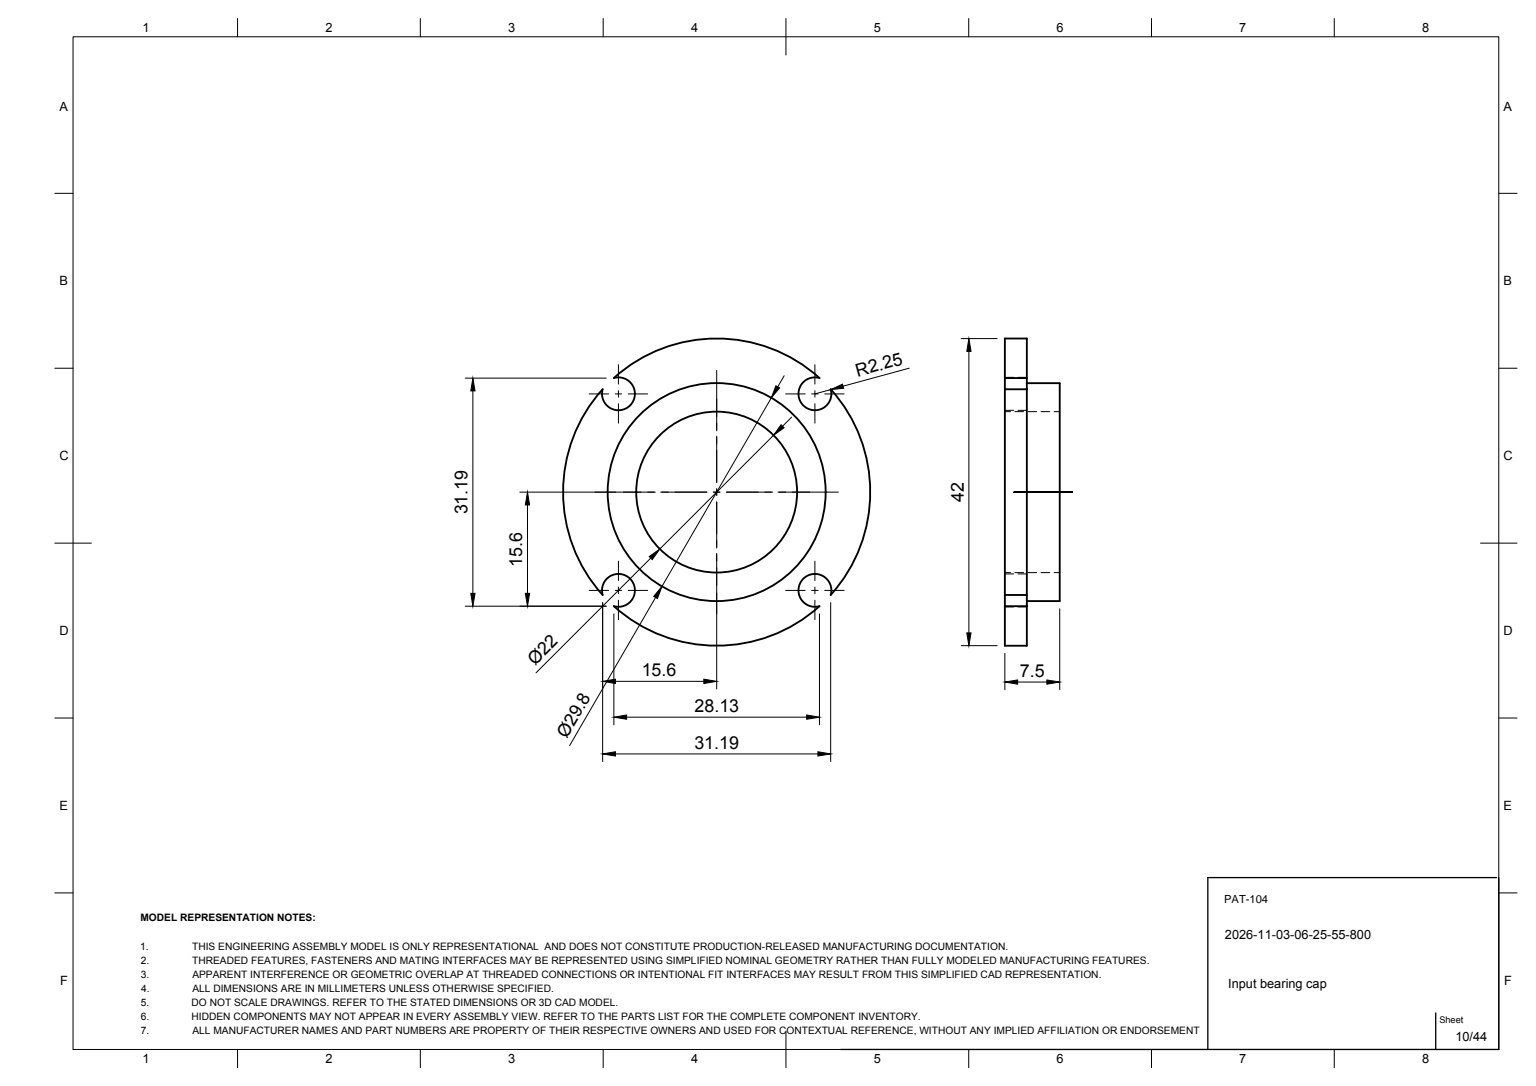
ISO-10303-21;
HEADER;
/* Generated by software containing ST-Developer
 * from STEP Tools, Inc. (www.steptools.com) 
 */

FILE_DESCRIPTION(
/* description */ ('Timing belt drive module 2 mm Pitch Timing 20T-40T'),

/* implementation_level */ '2;1');

FILE_NAME(
/* name */ 'Input bearing cap.step',
/* time_stamp */ '2026-10-28T03:25:12-07:00',
/* author */ (''),
/* organization */ (''),
/* preprocessor_version */ 'ST-DEVELOPER v20.2',
/* originating_system */ 'Autodesk Translation Framework v15.17.0.0',
/* authorisation */ '');

FILE_SCHEMA (('AUTOMOTIVE_DESIGN { 1 0 10303 214 3 1 1 }'));
ENDSEC;

DATA;
#10=MECHANICAL_DESIGN_GEOMETRIC_PRESENTATION_REPRESENTATION('',(#529),#17830);
#443=SHAPE_REPRESENTATION_RELATIONSHIP('SRR','None',#18013,#486);
#486=ADVANCED_BREP_SHAPE_REPRESENTATION('',(#587),#17788);
#529=STYLED_ITEM('',(#18317),#587);
#587=MANIFOLD_SOLID_BREP('Body1',#8986);
#667=FACE_BOUND('',#1583,.T.);
#668=FACE_BOUND('',#1590,.T.);
#669=FACE_BOUND('',#1593,.T.);
#815=PLANE('',#9651);
#816=PLANE('',#9668);
#817=PLANE('',#9671);
#1027=FACE_OUTER_BOUND('',#1578,.T.);
#1028=FACE_OUTER_BOUND('',#1579,.T.);
#1029=FACE_OUTER_BOUND('',#1580,.T.);
#1030=FACE_OUTER_BOUND('',#1581,.T.);
#1031=FACE_OUTER_BOUND('',#1582,.T.);
#1032=FACE_OUTER_BOUND('',#1584,.T.);
#1033=FACE_OUTER_BOUND('',#1585,.T.);
#1034=FACE_OUTER_BOUND('',#1586,.T.);
#1035=FACE_OUTER_BOUND('',#1587,.T.);
#1036=FACE_OUTER_BOUND('',#1588,.T.);
#1037=FACE_OUTER_BOUND('',#1589,.T.);
#1038=FACE_OUTER_BOUND('',#1591,.T.);
#1039=FACE_OUTER_BOUND('',#1592,.T.);
#1578=EDGE_LOOP('',(#6091,#6092,#6093,#6094));
#1579=EDGE_LOOP('',(#6095,#6096,#6097,#6098));
#1580=EDGE_LOOP('',(#6099,#6100,#6101,#6102));
#1581=EDGE_LOOP('',(#6103,#6104,#6105,#6106));
#1582=EDGE_LOOP('',(#6107,#6108,#6109,#6110,#6111,#6112,#6113,#6114));
#1583=EDGE_LOOP('',(#6115));
#1584=EDGE_LOOP('',(#6116,#6117,#6118,#6119));
#1585=EDGE_LOOP('',(#6120,#6121,#6122,#6123));
#1586=EDGE_LOOP('',(#6124,#6125,#6126,#6127));
#1587=EDGE_LOOP('',(#6128,#6129,#6130,#6131));
#1588=EDGE_LOOP('',(#6132,#6133,#6134,#6135));
#1589=EDGE_LOOP('',(#6136));
#1590=EDGE_LOOP('',(#6137));
#1591=EDGE_LOOP('',(#6138,#6139,#6140,#6141));
#1592=EDGE_LOOP('',(#6142,#6143,#6144,#6145,#6146,#6147,#6148,#6149));
#1593=EDGE_LOOP('',(#6150));
#2190=CIRCLE('',#9640,0.225);
#2191=CIRCLE('',#9641,0.225);
#2192=CIRCLE('',#9643,0.225);
#2193=CIRCLE('',#9644,0.225);
#2194=CIRCLE('',#9646,0.225);
#2195=CIRCLE('',#9647,0.225);
#2196=CIRCLE('',#9649,0.225);
#2197=CIRCLE('',#9650,0.225);
#2198=CIRCLE('',#9652,2.1);
#2199=CIRCLE('',#9653,2.1);
#2200=CIRCLE('',#9654,2.1);
#2201=CIRCLE('',#9655,2.1);
#2202=CIRCLE('',#9656,1.1);
#2203=CIRCLE('',#9658,2.1);
#2204=CIRCLE('',#9660,2.1);
#2205=CIRCLE('',#9662,2.1);
#2206=CIRCLE('',#9664,2.1);
#2207=CIRCLE('',#9666,1.49);
#2208=CIRCLE('',#9667,1.49);
#2209=CIRCLE('',#9669,1.1);
#2899=LINE('',#14214,#3377);
#2900=LINE('',#14218,#3378);
#2901=LINE('',#14223,#3379);
#2902=LINE('',#14227,#3380);
#2903=LINE('',#14232,#3381);
#2904=LINE('',#14236,#3382);
#2905=LINE('',#14241,#3383);
#2906=LINE('',#14245,#3384);
#2907=LINE('',#14266,#3385);
#2908=LINE('',#14272,#3386);
#3377=VECTOR('',#11166,1.);
#3378=VECTOR('',#11169,1.);
#3379=VECTOR('',#11174,1.);
#3380=VECTOR('',#11177,1.);
#3381=VECTOR('',#11182,1.);
#3382=VECTOR('',#11185,1.);
#3383=VECTOR('',#11190,1.);
#3384=VECTOR('',#11193,1.);
#3385=VECTOR('',#11228,1.49);
#3386=VECTOR('',#11237,1.1);
#3852=VERTEX_POINT('',#14212);
#3853=VERTEX_POINT('',#14213);
#3854=VERTEX_POINT('',#14215);
#3855=VERTEX_POINT('',#14217);
#3856=VERTEX_POINT('',#14221);
#3857=VERTEX_POINT('',#14222);
#3858=VERTEX_POINT('',#14224);
#3859=VERTEX_POINT('',#14226);
#3860=VERTEX_POINT('',#14230);
#3861=VERTEX_POINT('',#14231);
#3862=VERTEX_POINT('',#14233);
#3863=VERTEX_POINT('',#14235);
#3864=VERTEX_POINT('',#14239);
#3865=VERTEX_POINT('',#14240);
#3866=VERTEX_POINT('',#14242);
#3867=VERTEX_POINT('',#14244);
#3868=VERTEX_POINT('',#14252);
#3869=VERTEX_POINT('',#14263);
#3870=VERTEX_POINT('',#14265);
#3871=VERTEX_POINT('',#14269);
#4728=EDGE_CURVE('',#3852,#3853,#2899,.T.);
#4729=EDGE_CURVE('',#3854,#3852,#2190,.T.);
#4730=EDGE_CURVE('',#3855,#3854,#2900,.T.);
#4731=EDGE_CURVE('',#3853,#3855,#2191,.T.);
#4732=EDGE_CURVE('',#3856,#3857,#2901,.T.);
#4733=EDGE_CURVE('',#3858,#3856,#2192,.T.);
#4734=EDGE_CURVE('',#3859,#3858,#2902,.T.);
#4735=EDGE_CURVE('',#3857,#3859,#2193,.T.);
#4736=EDGE_CURVE('',#3860,#3861,#2903,.T.);
#4737=EDGE_CURVE('',#3862,#3860,#2194,.T.);
#4738=EDGE_CURVE('',#3863,#3862,#2904,.T.);
#4739=EDGE_CURVE('',#3861,#3863,#2195,.T.);
#4740=EDGE_CURVE('',#3864,#3865,#2905,.T.);
#4741=EDGE_CURVE('',#3866,#3864,#2196,.T.);
#4742=EDGE_CURVE('',#3867,#3866,#2906,.T.);
#4743=EDGE_CURVE('',#3865,#3867,#2197,.T.);
#4744=EDGE_CURVE('',#3866,#3852,#2198,.T.);
#4745=EDGE_CURVE('',#3862,#3864,#2199,.T.);
#4746=EDGE_CURVE('',#3858,#3860,#2200,.T.);
#4747=EDGE_CURVE('',#3854,#3856,#2201,.T.);
#4748=EDGE_CURVE('',#3868,#3868,#2202,.T.);
#4749=EDGE_CURVE('',#3863,#3865,#2203,.T.);
#4750=EDGE_CURVE('',#3859,#3861,#2204,.T.);
#4751=EDGE_CURVE('',#3867,#3853,#2205,.T.);
#4752=EDGE_CURVE('',#3855,#3857,#2206,.T.);
#4753=EDGE_CURVE('',#3869,#3869,#2207,.T.);
#4754=EDGE_CURVE('',#3869,#3870,#2907,.T.);
#4755=EDGE_CURVE('',#3870,#3870,#2208,.T.);
#4756=EDGE_CURVE('',#3871,#3871,#2209,.T.);
#4757=EDGE_CURVE('',#3871,#3868,#2908,.T.);
#6091=ORIENTED_EDGE('',*,*,#4728,.F.);
#6092=ORIENTED_EDGE('',*,*,#4729,.F.);
#6093=ORIENTED_EDGE('',*,*,#4730,.F.);
#6094=ORIENTED_EDGE('',*,*,#4731,.F.);
#6095=ORIENTED_EDGE('',*,*,#4732,.F.);
#6096=ORIENTED_EDGE('',*,*,#4733,.F.);
#6097=ORIENTED_EDGE('',*,*,#4734,.F.);
#6098=ORIENTED_EDGE('',*,*,#4735,.F.);
#6099=ORIENTED_EDGE('',*,*,#4736,.F.);
#6100=ORIENTED_EDGE('',*,*,#4737,.F.);
#6101=ORIENTED_EDGE('',*,*,#4738,.F.);
#6102=ORIENTED_EDGE('',*,*,#4739,.F.);
#6103=ORIENTED_EDGE('',*,*,#4740,.F.);
#6104=ORIENTED_EDGE('',*,*,#4741,.F.);
#6105=ORIENTED_EDGE('',*,*,#4742,.F.);
#6106=ORIENTED_EDGE('',*,*,#4743,.F.);
#6107=ORIENTED_EDGE('',*,*,#4729,.T.);
#6108=ORIENTED_EDGE('',*,*,#4744,.F.);
#6109=ORIENTED_EDGE('',*,*,#4741,.T.);
#6110=ORIENTED_EDGE('',*,*,#4745,.F.);
#6111=ORIENTED_EDGE('',*,*,#4737,.T.);
#6112=ORIENTED_EDGE('',*,*,#4746,.F.);
#6113=ORIENTED_EDGE('',*,*,#4733,.T.);
#6114=ORIENTED_EDGE('',*,*,#4747,.F.);
#6115=ORIENTED_EDGE('',*,*,#4748,.F.);
#6116=ORIENTED_EDGE('',*,*,#4738,.T.);
#6117=ORIENTED_EDGE('',*,*,#4745,.T.);
#6118=ORIENTED_EDGE('',*,*,#4740,.T.);
#6119=ORIENTED_EDGE('',*,*,#4749,.F.);
#6120=ORIENTED_EDGE('',*,*,#4734,.T.);
#6121=ORIENTED_EDGE('',*,*,#4746,.T.);
#6122=ORIENTED_EDGE('',*,*,#4736,.T.);
#6123=ORIENTED_EDGE('',*,*,#4750,.F.);
#6124=ORIENTED_EDGE('',*,*,#4728,.T.);
#6125=ORIENTED_EDGE('',*,*,#4751,.F.);
#6126=ORIENTED_EDGE('',*,*,#4742,.T.);
#6127=ORIENTED_EDGE('',*,*,#4744,.T.);
#6128=ORIENTED_EDGE('',*,*,#4730,.T.);
#6129=ORIENTED_EDGE('',*,*,#4747,.T.);
#6130=ORIENTED_EDGE('',*,*,#4732,.T.);
#6131=ORIENTED_EDGE('',*,*,#4752,.F.);
#6132=ORIENTED_EDGE('',*,*,#4753,.F.);
#6133=ORIENTED_EDGE('',*,*,#4754,.T.);
#6134=ORIENTED_EDGE('',*,*,#4755,.F.);
#6135=ORIENTED_EDGE('',*,*,#4754,.F.);
#6136=ORIENTED_EDGE('',*,*,#4753,.T.);
#6137=ORIENTED_EDGE('',*,*,#4756,.T.);
#6138=ORIENTED_EDGE('',*,*,#4756,.F.);
#6139=ORIENTED_EDGE('',*,*,#4757,.T.);
#6140=ORIENTED_EDGE('',*,*,#4748,.T.);
#6141=ORIENTED_EDGE('',*,*,#4757,.F.);
#6142=ORIENTED_EDGE('',*,*,#4731,.T.);
#6143=ORIENTED_EDGE('',*,*,#4752,.T.);
#6144=ORIENTED_EDGE('',*,*,#4735,.T.);
#6145=ORIENTED_EDGE('',*,*,#4750,.T.);
#6146=ORIENTED_EDGE('',*,*,#4739,.T.);
#6147=ORIENTED_EDGE('',*,*,#4749,.T.);
#6148=ORIENTED_EDGE('',*,*,#4743,.T.);
#6149=ORIENTED_EDGE('',*,*,#4751,.T.);
#6150=ORIENTED_EDGE('',*,*,#4755,.T.);
#8204=CYLINDRICAL_SURFACE('',#9639,0.225);
#8205=CYLINDRICAL_SURFACE('',#9642,0.225);
#8206=CYLINDRICAL_SURFACE('',#9645,0.225);
#8207=CYLINDRICAL_SURFACE('',#9648,0.225);
#8208=CYLINDRICAL_SURFACE('',#9657,2.1);
#8209=CYLINDRICAL_SURFACE('',#9659,2.1);
#8210=CYLINDRICAL_SURFACE('',#9661,2.1);
#8211=CYLINDRICAL_SURFACE('',#9663,2.1);
#8212=CYLINDRICAL_SURFACE('',#9665,1.49);
#8213=CYLINDRICAL_SURFACE('',#9670,1.1);
#8525=ADVANCED_FACE('',(#1027),#8204,.F.);
#8526=ADVANCED_FACE('',(#1028),#8205,.F.);
#8527=ADVANCED_FACE('',(#1029),#8206,.F.);
#8528=ADVANCED_FACE('',(#1030),#8207,.F.);
#8529=ADVANCED_FACE('',(#1031,#667),#815,.F.);
#8530=ADVANCED_FACE('',(#1032),#8208,.T.);
#8531=ADVANCED_FACE('',(#1033),#8209,.T.);
#8532=ADVANCED_FACE('',(#1034),#8210,.T.);
#8533=ADVANCED_FACE('',(#1035),#8211,.T.);
#8534=ADVANCED_FACE('',(#1036),#8212,.T.);
#8535=ADVANCED_FACE('',(#1037,#668),#816,.T.);
#8536=ADVANCED_FACE('',(#1038),#8213,.F.);
#8537=ADVANCED_FACE('',(#1039,#669),#817,.T.);
#8986=CLOSED_SHELL('',(#8525,#8526,#8527,#8528,#8529,#8530,#8531,#8532,
#8533,#8534,#8535,#8536,#8537));
#9638=AXIS2_PLACEMENT_3D('',#14210,#11162,#11163);
#9639=AXIS2_PLACEMENT_3D('',#14211,#11164,#11165);
#9640=AXIS2_PLACEMENT_3D('',#14216,#11167,#11168);
#9641=AXIS2_PLACEMENT_3D('',#14219,#11170,#11171);
#9642=AXIS2_PLACEMENT_3D('',#14220,#11172,#11173);
#9643=AXIS2_PLACEMENT_3D('',#14225,#11175,#11176);
#9644=AXIS2_PLACEMENT_3D('',#14228,#11178,#11179);
#9645=AXIS2_PLACEMENT_3D('',#14229,#11180,#11181);
#9646=AXIS2_PLACEMENT_3D('',#14234,#11183,#11184);
#9647=AXIS2_PLACEMENT_3D('',#14237,#11186,#11187);
#9648=AXIS2_PLACEMENT_3D('',#14238,#11188,#11189);
#9649=AXIS2_PLACEMENT_3D('',#14243,#11191,#11192);
#9650=AXIS2_PLACEMENT_3D('',#14246,#11194,#11195);
#9651=AXIS2_PLACEMENT_3D('',#14247,#11196,#11197);
#9652=AXIS2_PLACEMENT_3D('',#14248,#11198,#11199);
#9653=AXIS2_PLACEMENT_3D('',#14249,#11200,#11201);
#9654=AXIS2_PLACEMENT_3D('',#14250,#11202,#11203);
#9655=AXIS2_PLACEMENT_3D('',#14251,#11204,#11205);
#9656=AXIS2_PLACEMENT_3D('',#14253,#11206,#11207);
#9657=AXIS2_PLACEMENT_3D('',#14254,#11208,#11209);
#9658=AXIS2_PLACEMENT_3D('',#14255,#11210,#11211);
#9659=AXIS2_PLACEMENT_3D('',#14256,#11212,#11213);
#9660=AXIS2_PLACEMENT_3D('',#14257,#11214,#11215);
#9661=AXIS2_PLACEMENT_3D('',#14258,#11216,#11217);
#9662=AXIS2_PLACEMENT_3D('',#14259,#11218,#11219);
#9663=AXIS2_PLACEMENT_3D('',#14260,#11220,#11221);
#9664=AXIS2_PLACEMENT_3D('',#14261,#11222,#11223);
#9665=AXIS2_PLACEMENT_3D('',#14262,#11224,#11225);
#9666=AXIS2_PLACEMENT_3D('',#14264,#11226,#11227);
#9667=AXIS2_PLACEMENT_3D('',#14267,#11229,#11230);
#9668=AXIS2_PLACEMENT_3D('',#14268,#11231,#11232);
#9669=AXIS2_PLACEMENT_3D('',#14270,#11233,#11234);
#9670=AXIS2_PLACEMENT_3D('',#14271,#11235,#11236);
#9671=AXIS2_PLACEMENT_3D('',#14273,#11238,#11239);
#11162=DIRECTION('axis',(0.,0.,1.));
#11163=DIRECTION('refdir',(1.,0.,0.));
#11164=DIRECTION('center_axis',(0.,1.,0.));
#11165=DIRECTION('ref_axis',(0.707106781186546,0.,0.707106781186549));
#11166=DIRECTION('',(0.,1.,0.));
#11167=DIRECTION('center_axis',(0.,1.,0.));
#11168=DIRECTION('ref_axis',(1.,0.,0.));
#11169=DIRECTION('',(0.,-1.,0.));
#11170=DIRECTION('center_axis',(0.,-1.,0.));
#11171=DIRECTION('ref_axis',(1.,0.,0.));
#11172=DIRECTION('center_axis',(0.,1.,0.));
#11173=DIRECTION('ref_axis',(0.707106781186547,0.,-0.707106781186548));
#11174=DIRECTION('',(0.,1.,0.));
#11175=DIRECTION('center_axis',(0.,1.,0.));
#11176=DIRECTION('ref_axis',(1.,0.,0.));
#11177=DIRECTION('',(0.,-1.,0.));
#11178=DIRECTION('center_axis',(0.,-1.,0.));
#11179=DIRECTION('ref_axis',(1.,0.,0.));
#11180=DIRECTION('center_axis',(0.,1.,0.));
#11181=DIRECTION('ref_axis',(-0.707106781186552,0.,-0.707106781186543));
#11182=DIRECTION('',(0.,1.,0.));
#11183=DIRECTION('center_axis',(0.,1.,0.));
#11184=DIRECTION('ref_axis',(1.,0.,0.));
#11185=DIRECTION('',(0.,-1.,0.));
#11186=DIRECTION('center_axis',(0.,-1.,0.));
#11187=DIRECTION('ref_axis',(1.,0.,0.));
#11188=DIRECTION('center_axis',(0.,1.,0.));
#11189=DIRECTION('ref_axis',(-0.707106781186546,0.,0.707106781186549));
#11190=DIRECTION('',(0.,1.,0.));
#11191=DIRECTION('center_axis',(0.,1.,0.));
#11192=DIRECTION('ref_axis',(1.,0.,0.));
#11193=DIRECTION('',(0.,-1.,0.));
#11194=DIRECTION('center_axis',(0.,-1.,0.));
#11195=DIRECTION('ref_axis',(1.,0.,0.));
#11196=DIRECTION('center_axis',(0.,1.,0.));
#11197=DIRECTION('ref_axis',(1.,0.,0.));
#11198=DIRECTION('center_axis',(0.,1.,0.));
#11199=DIRECTION('ref_axis',(1.,0.,0.));
#11200=DIRECTION('center_axis',(0.,1.,0.));
#11201=DIRECTION('ref_axis',(1.,0.,0.));
#11202=DIRECTION('center_axis',(0.,1.,0.));
#11203=DIRECTION('ref_axis',(1.,0.,0.));
#11204=DIRECTION('center_axis',(0.,1.,0.));
#11205=DIRECTION('ref_axis',(1.,0.,0.));
#11206=DIRECTION('center_axis',(0.,-1.,0.));
#11207=DIRECTION('ref_axis',(1.,0.,0.));
#11208=DIRECTION('center_axis',(0.,1.,0.));
#11209=DIRECTION('ref_axis',(1.,0.,0.));
#11210=DIRECTION('center_axis',(0.,1.,0.));
#11211=DIRECTION('ref_axis',(1.,0.,0.));
#11212=DIRECTION('center_axis',(0.,1.,0.));
#11213=DIRECTION('ref_axis',(1.,0.,0.));
#11214=DIRECTION('center_axis',(0.,1.,0.));
#11215=DIRECTION('ref_axis',(1.,0.,0.));
#11216=DIRECTION('center_axis',(0.,1.,0.));
#11217=DIRECTION('ref_axis',(1.,0.,0.));
#11218=DIRECTION('center_axis',(0.,1.,0.));
#11219=DIRECTION('ref_axis',(1.,0.,0.));
#11220=DIRECTION('center_axis',(0.,1.,0.));
#11221=DIRECTION('ref_axis',(-1.,0.,-1.22464679914735E-16));
#11222=DIRECTION('center_axis',(0.,1.,0.));
#11223=DIRECTION('ref_axis',(1.,0.,0.));
#11224=DIRECTION('center_axis',(0.,1.,0.));
#11225=DIRECTION('ref_axis',(1.,0.,0.));
#11226=DIRECTION('center_axis',(0.,1.,0.));
#11227=DIRECTION('ref_axis',(1.,0.,0.));
#11228=DIRECTION('',(0.,-1.,0.));
#11229=DIRECTION('center_axis',(0.,-1.,0.));
#11230=DIRECTION('ref_axis',(1.,0.,0.));
#11231=DIRECTION('center_axis',(0.,1.,0.));
#11232=DIRECTION('ref_axis',(1.,0.,0.));
#11233=DIRECTION('center_axis',(0.,-1.,0.));
#11234=DIRECTION('ref_axis',(1.,0.,0.));
#11235=DIRECTION('center_axis',(0.,1.,0.));
#11236=DIRECTION('ref_axis',(1.,0.,0.));
#11237=DIRECTION('',(0.,-1.,0.));
#11238=DIRECTION('center_axis',(0.,1.,0.));
#11239=DIRECTION('ref_axis',(1.,0.,0.));
#14210=CARTESIAN_POINT('',(0.,0.,0.));
#14211=CARTESIAN_POINT('Origin',(-1.34350288425444,-2.2,5.65649711574556));
#14212=CARTESIAN_POINT('',(-1.40634555589641,-2.1,5.4404512904656));
#14213=CARTESIAN_POINT('',(-1.40634555589641,-1.8,5.4404512904656));
#14214=CARTESIAN_POINT('',(-1.40634555589641,-2.2,5.4404512904656));
#14215=CARTESIAN_POINT('',(-1.5595487095344,-2.1,5.59365444410359));
#14216=CARTESIAN_POINT('Origin',(-1.34350288425444,-2.1,5.65649711574556));
#14217=CARTESIAN_POINT('',(-1.5595487095344,-1.8,5.59365444410359));
#14218=CARTESIAN_POINT('',(-1.5595487095344,-2.2,5.59365444410359));
#14219=CARTESIAN_POINT('Origin',(-1.34350288425444,-1.8,5.65649711574556));
#14220=CARTESIAN_POINT('Origin',(-1.34350288425444,-2.2,8.34350288425444));
#14221=CARTESIAN_POINT('',(-1.5595487095344,-2.1,8.40634555589641));
#14222=CARTESIAN_POINT('',(-1.5595487095344,-1.8,8.40634555589641));
#14223=CARTESIAN_POINT('',(-1.5595487095344,-2.2,8.40634555589641));
#14224=CARTESIAN_POINT('',(-1.40634555589641,-2.1,8.5595487095344));
#14225=CARTESIAN_POINT('Origin',(-1.34350288425444,-2.1,8.34350288425444));
#14226=CARTESIAN_POINT('',(-1.40634555589641,-1.8,8.5595487095344));
#14227=CARTESIAN_POINT('',(-1.40634555589641,-2.2,8.5595487095344));
#14228=CARTESIAN_POINT('Origin',(-1.34350288425444,-1.8,8.34350288425444));
#14229=CARTESIAN_POINT('Origin',(1.34350288425444,-2.2,8.34350288425444));
#14230=CARTESIAN_POINT('',(1.40634555589641,-2.1,8.5595487095344));
#14231=CARTESIAN_POINT('',(1.40634555589641,-1.8,8.5595487095344));
#14232=CARTESIAN_POINT('',(1.40634555589641,-2.2,8.5595487095344));
#14233=CARTESIAN_POINT('',(1.5595487095344,-2.1,8.40634555589641));
#14234=CARTESIAN_POINT('Origin',(1.34350288425444,-2.1,8.34350288425444));
#14235=CARTESIAN_POINT('',(1.5595487095344,-1.8,8.40634555589641));
#14236=CARTESIAN_POINT('',(1.5595487095344,-2.2,8.40634555589641));
#14237=CARTESIAN_POINT('Origin',(1.34350288425444,-1.8,8.34350288425444));
#14238=CARTESIAN_POINT('Origin',(1.34350288425444,-2.2,5.65649711574556));
#14239=CARTESIAN_POINT('',(1.5595487095344,-2.1,5.59365444410359));
#14240=CARTESIAN_POINT('',(1.5595487095344,-1.8,5.59365444410359));
#14241=CARTESIAN_POINT('',(1.5595487095344,-2.2,5.59365444410359));
#14242=CARTESIAN_POINT('',(1.40634555589641,-2.1,5.4404512904656));
#14243=CARTESIAN_POINT('Origin',(1.34350288425444,-2.1,5.65649711574556));
#14244=CARTESIAN_POINT('',(1.40634555589641,-1.8,5.4404512904656));
#14245=CARTESIAN_POINT('',(1.40634555589641,-2.2,5.4404512904656));
#14246=CARTESIAN_POINT('Origin',(1.34350288425444,-1.8,5.65649711574556));
#14247=CARTESIAN_POINT('Origin',(0.,-2.1,7.));
#14248=CARTESIAN_POINT('Origin',(0.,-2.1,7.));
#14249=CARTESIAN_POINT('Origin',(0.,-2.1,7.));
#14250=CARTESIAN_POINT('Origin',(0.,-2.1,7.));
#14251=CARTESIAN_POINT('Origin',(0.,-2.1,7.));
#14252=CARTESIAN_POINT('',(-1.1,-2.1,7.));
#14253=CARTESIAN_POINT('Origin',(0.,-2.1,7.));
#14254=CARTESIAN_POINT('Origin',(0.,-2.1,7.));
#14255=CARTESIAN_POINT('Origin',(0.,-1.8,7.));
#14256=CARTESIAN_POINT('Origin',(0.,-2.1,7.));
#14257=CARTESIAN_POINT('Origin',(0.,-1.8,7.));
#14258=CARTESIAN_POINT('Origin',(0.,-2.1,7.));
#14259=CARTESIAN_POINT('Origin',(0.,-1.8,7.));
#14260=CARTESIAN_POINT('Origin',(0.,-2.1,7.));
#14261=CARTESIAN_POINT('Origin',(0.,-1.8,7.));
#14262=CARTESIAN_POINT('Origin',(0.,-1.8,7.));
#14263=CARTESIAN_POINT('',(-1.49,-1.35,7.));
#14264=CARTESIAN_POINT('Origin',(0.,-1.35,7.));
#14265=CARTESIAN_POINT('',(-1.49,-1.8,7.));
#14266=CARTESIAN_POINT('',(-1.49,-1.8,7.));
#14267=CARTESIAN_POINT('Origin',(0.,-1.8,7.));
#14268=CARTESIAN_POINT('Origin',(0.,-1.35,7.));
#14269=CARTESIAN_POINT('',(-1.1,-1.35,7.));
#14270=CARTESIAN_POINT('Origin',(0.,-1.35,7.));
#14271=CARTESIAN_POINT('Origin',(0.,-2.1,7.));
#14272=CARTESIAN_POINT('',(-1.1,-2.1,7.));
#14273=CARTESIAN_POINT('Origin',(0.,-1.8,7.));
#17738=UNCERTAINTY_MEASURE_WITH_UNIT(LENGTH_MEASURE(0.001),#17831,
'DISTANCE_ACCURACY_VALUE',
'Maximum model space distance between geometric entities at asserted c
onnectivities');
#17780=UNCERTAINTY_MEASURE_WITH_UNIT(LENGTH_MEASURE(0.001),#17831,
'DISTANCE_ACCURACY_VALUE',
'Maximum model space distance between geometric entities at asserted c
onnectivities');
#17788=(
GEOMETRIC_REPRESENTATION_CONTEXT(3)
GLOBAL_UNCERTAINTY_ASSIGNED_CONTEXT((#17738))
GLOBAL_UNIT_ASSIGNED_CONTEXT((#17831,#17833,#17834))
REPRESENTATION_CONTEXT('','3D')
);
#17830=(
GEOMETRIC_REPRESENTATION_CONTEXT(3)
GLOBAL_UNCERTAINTY_ASSIGNED_CONTEXT((#17780))
GLOBAL_UNIT_ASSIGNED_CONTEXT((#17831,#17833,#17834))
REPRESENTATION_CONTEXT('','3D')
);
#17831=(
LENGTH_UNIT()
NAMED_UNIT(*)
SI_UNIT(.CENTI.,.METRE.)
);
#17833=(
NAMED_UNIT(*)
PLANE_ANGLE_UNIT()
SI_UNIT($,.RADIAN.)
);
#17834=(
NAMED_UNIT(*)
SI_UNIT($,.STERADIAN.)
SOLID_ANGLE_UNIT()
);
#17842=SHAPE_DEFINITION_REPRESENTATION(#17891,#18013);
#17891=PRODUCT_DEFINITION_SHAPE('',$,#18063);
#18013=SHAPE_REPRESENTATION('',(#9638),#17788);
#18055=PRODUCT_DEFINITION_CONTEXT('part definition',#18204,'design');
#18063=PRODUCT_DEFINITION('Input bearing cap','Input bearing cap',#18112,
#18055);
#18112=PRODUCT_DEFINITION_FORMATION('',$,#18213);
#18204=APPLICATION_CONTEXT(
'Core Data for Automotive Mechanical Design Process');
#18205=PRODUCT_CONTEXT('part definition',#18204,'mechanical');
#18213=PRODUCT('Input bearing cap','Input bearing cap',
'Input bearing cap',(#18205));
#18311=COLOUR_RGB('Grey',0.48,0.52,0.57);
#18312=FILL_AREA_STYLE_COLOUR('',#18311);
#18313=FILL_AREA_STYLE('',(#18312));
#18314=SURFACE_STYLE_FILL_AREA(#18313);
#18315=SURFACE_SIDE_STYLE('',(#18314));
#18316=SURFACE_STYLE_USAGE(.BOTH.,#18315);
#18317=PRESENTATION_STYLE_ASSIGNMENT((#18316));
ENDSEC;
END-ISO-10303-21;
